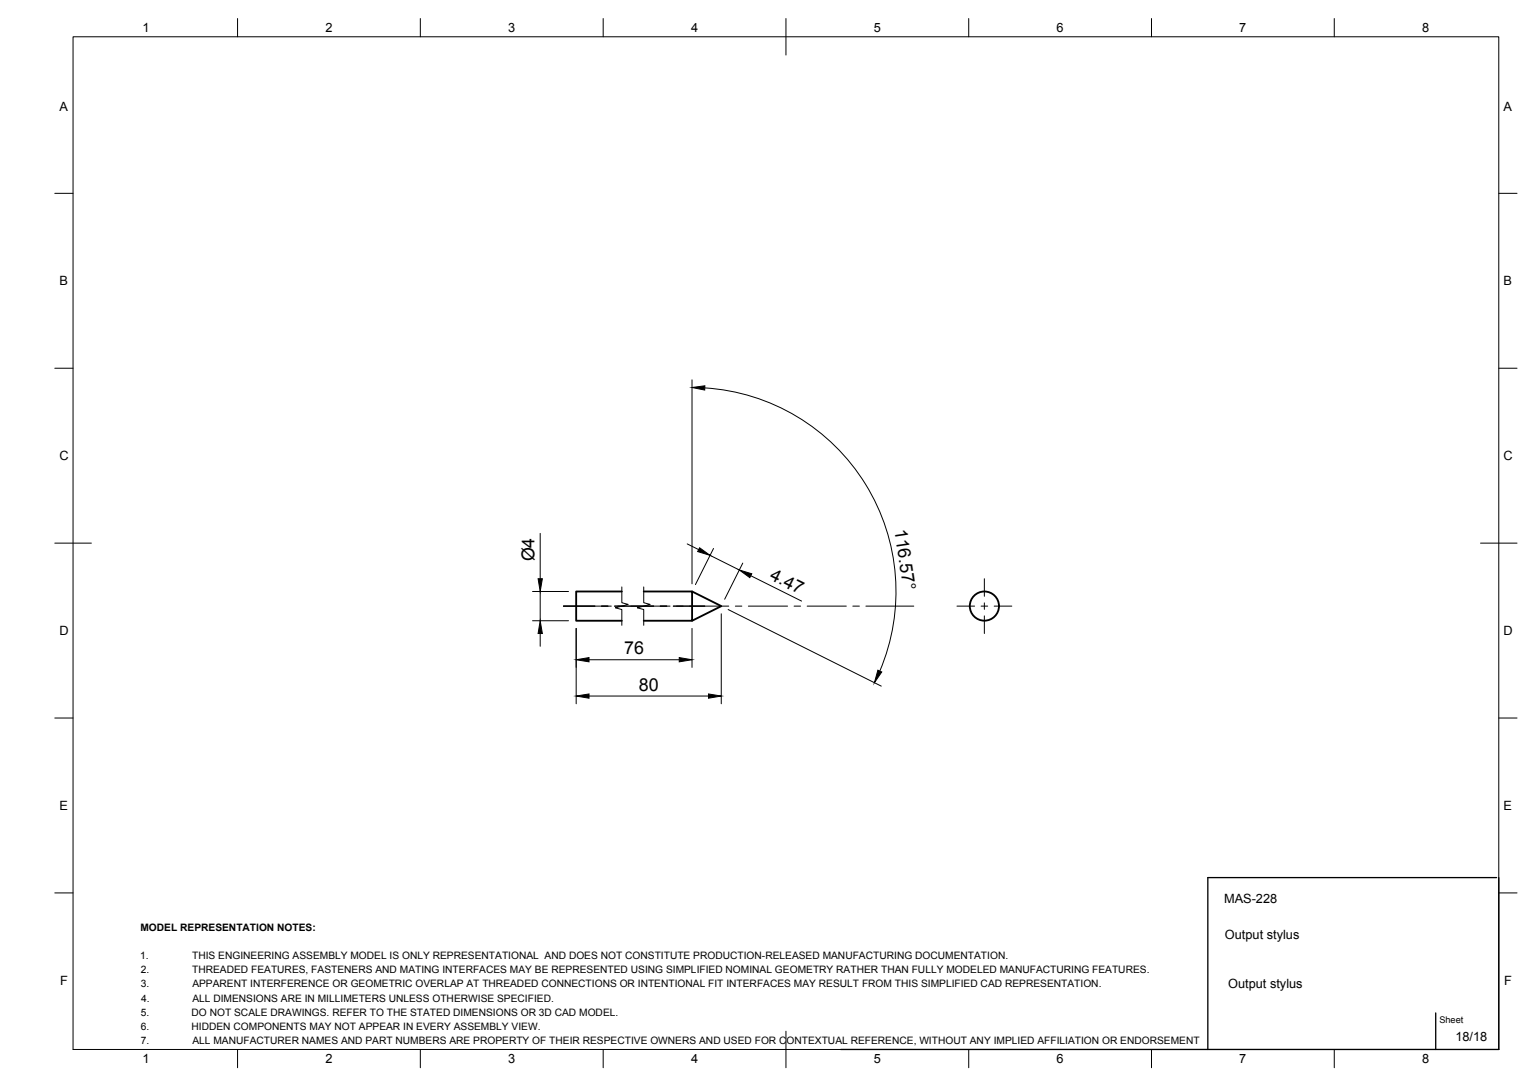
ISO-10303-21;
HEADER;
/* Generated by software containing ST-Developer
 * from STEP Tools, Inc. (www.steptools.com) 
 */

FILE_DESCRIPTION(
/* description */ ('Independent Peaucellier-Lipkin straight-line linkage. Radius arms 100
 mm, inversion-cell links 60 mm, crank radius and fixed-pivot spacing 
32 mm. Inversion constant 6400 mm squared, nominal output straight lin
e X=100 mm. Overhead bearing bridge clears the layered moving links. N
o accuracy or load rating assigned.'),
/* implementation_level */ '2;1');

FILE_NAME(
/* name */ 'Output stylus.step',
/* time_stamp */ '2026-11-09T18:06:16-08:00',
/* author */ (''),
/* organization */ (''),
/* preprocessor_version */ 'ST-DEVELOPER v20.2',
/* originating_system */ 'Autodesk Translation Framework v15.17.0.0',
/* authorisation */ '');

FILE_SCHEMA (('AUTOMOTIVE_DESIGN { 1 0 10303 214 3 1 1 }'));
ENDSEC;

DATA;
#10=MECHANICAL_DESIGN_GEOMETRIC_PRESENTATION_REPRESENTATION('',(#294),#3581);
#247=CONICAL_SURFACE('',#2252,1.,0.463647609000806);
#260=SHAPE_REPRESENTATION_RELATIONSHIP('SRR','None',#3694,#277);
#277=ADVANCED_BREP_SHAPE_REPRESENTATION('',(#311),#3576);
#294=STYLED_ITEM('',(#3785),#311);
#311=MANIFOLD_SOLID_BREP('Body1',#1880);
#411=PLANE('',#2251);
#510=FACE_OUTER_BOUND('',#662,.T.);
#511=FACE_OUTER_BOUND('',#663,.T.);
#512=FACE_OUTER_BOUND('',#664,.T.);
#662=EDGE_LOOP('',(#1628,#1629,#1630,#1631));
#663=EDGE_LOOP('',(#1632));
#664=EDGE_LOOP('',(#1633,#1634,#1635));
#775=LINE('',#3392,#873);
#776=LINE('',#3397,#874);
#873=VECTOR('',#2793,2.);
#874=VECTOR('',#2800,1.);
#967=CIRCLE('',#2249,2.);
#968=CIRCLE('',#2250,2.);
#1093=VERTEX_POINT('',#3389);
#1094=VERTEX_POINT('',#3391);
#1095=VERTEX_POINT('',#3396);
#1276=EDGE_CURVE('',#1093,#1093,#967,.T.);
#1277=EDGE_CURVE('',#1093,#1094,#775,.T.);
#1278=EDGE_CURVE('',#1094,#1094,#968,.T.);
#1279=EDGE_CURVE('',#1094,#1095,#776,.T.);
#1628=ORIENTED_EDGE('',*,*,#1276,.F.);
#1629=ORIENTED_EDGE('',*,*,#1277,.T.);
#1630=ORIENTED_EDGE('',*,*,#1278,.T.);
#1631=ORIENTED_EDGE('',*,*,#1277,.F.);
#1632=ORIENTED_EDGE('',*,*,#1276,.T.);
#1633=ORIENTED_EDGE('',*,*,#1278,.F.);
#1634=ORIENTED_EDGE('',*,*,#1279,.T.);
#1635=ORIENTED_EDGE('',*,*,#1279,.F.);
#1746=CYLINDRICAL_SURFACE('',#2248,2.);
#1842=ADVANCED_FACE('',(#510),#1746,.T.);
#1843=ADVANCED_FACE('',(#511),#411,.T.);
#1844=ADVANCED_FACE('',(#512),#247,.T.);
#1880=CLOSED_SHELL('',(#1842,#1843,#1844));
#2247=AXIS2_PLACEMENT_3D('',#3387,#2787,#2788);
#2248=AXIS2_PLACEMENT_3D('',#3388,#2789,#2790);
#2249=AXIS2_PLACEMENT_3D('',#3390,#2791,#2792);
#2250=AXIS2_PLACEMENT_3D('',#3393,#2794,#2795);
#2251=AXIS2_PLACEMENT_3D('',#3394,#2796,#2797);
#2252=AXIS2_PLACEMENT_3D('',#3395,#2798,#2799);
#2787=DIRECTION('axis',(0.,0.,1.));
#2788=DIRECTION('refdir',(1.,0.,0.));
#2789=DIRECTION('center_axis',(0.,0.,1.));
#2790=DIRECTION('ref_axis',(1.,0.,0.));
#2791=DIRECTION('center_axis',(0.,0.,1.));
#2792=DIRECTION('ref_axis',(1.,0.,0.));
#2793=DIRECTION('',(0.,0.,-1.));
#2794=DIRECTION('center_axis',(0.,0.,1.));
#2795=DIRECTION('ref_axis',(1.,0.,0.));
#2796=DIRECTION('center_axis',(0.,0.,1.));
#2797=DIRECTION('ref_axis',(1.,0.,0.));
#2798=DIRECTION('center_axis',(0.,0.,1.));
#2799=DIRECTION('ref_axis',(1.,0.,0.));
#2800=DIRECTION('',(0.447213595499958,5.47678698264203E-17,-0.894427190999916));
#3387=CARTESIAN_POINT('',(0.,0.,0.));
#3388=CARTESIAN_POINT('Origin',(0.,0.,4.));
#3389=CARTESIAN_POINT('',(-2.,-2.44929359829471E-16,80.));
#3390=CARTESIAN_POINT('Origin',(0.,0.,80.));
#3391=CARTESIAN_POINT('',(-2.,-2.44929359829471E-16,4.));
#3392=CARTESIAN_POINT('',(-2.,-2.44929359829471E-16,4.));
#3393=CARTESIAN_POINT('Origin',(0.,0.,4.));
#3394=CARTESIAN_POINT('Origin',(0.,0.,80.));
#3395=CARTESIAN_POINT('Origin',(0.,0.,2.));
#3396=CARTESIAN_POINT('',(0.,0.,0.));
#3397=CARTESIAN_POINT('',(-1.,-1.22464679914735E-16,2.));
#3557=UNCERTAINTY_MEASURE_WITH_UNIT(LENGTH_MEASURE(0.01),#3582,
'DISTANCE_ACCURACY_VALUE',
'Maximum model space distance between geometric entities at asserted c
onnectivities');
#3562=UNCERTAINTY_MEASURE_WITH_UNIT(LENGTH_MEASURE(0.01),#3582,
'DISTANCE_ACCURACY_VALUE',
'Maximum model space distance between geometric entities at asserted c
onnectivities');
#3576=(
GEOMETRIC_REPRESENTATION_CONTEXT(3)
GLOBAL_UNCERTAINTY_ASSIGNED_CONTEXT((#3557))
GLOBAL_UNIT_ASSIGNED_CONTEXT((#3582,#3584,#3585))
REPRESENTATION_CONTEXT('','3D')
);
#3581=(
GEOMETRIC_REPRESENTATION_CONTEXT(3)
GLOBAL_UNCERTAINTY_ASSIGNED_CONTEXT((#3562))
GLOBAL_UNIT_ASSIGNED_CONTEXT((#3582,#3584,#3585))
REPRESENTATION_CONTEXT('','3D')
);
#3582=(
LENGTH_UNIT()
NAMED_UNIT(*)
SI_UNIT(.MILLI.,.METRE.)
);
#3584=(
NAMED_UNIT(*)
PLANE_ANGLE_UNIT()
SI_UNIT($,.RADIAN.)
);
#3585=(
NAMED_UNIT(*)
SI_UNIT($,.STERADIAN.)
SOLID_ANGLE_UNIT()
);
#3599=SHAPE_DEFINITION_REPRESENTATION(#3617,#3694);
#3617=PRODUCT_DEFINITION_SHAPE('',$,#3713);
#3694=SHAPE_REPRESENTATION('',(#2247),#3576);
#3699=PRODUCT_DEFINITION_CONTEXT('part definition',#3755,'design');
#3713=PRODUCT_DEFINITION('Output stylus','Output stylus',#3731,#3699);
#3731=PRODUCT_DEFINITION_FORMATION('',$,#3770);
#3755=APPLICATION_CONTEXT(
'Core Data for Automotive Mechanical Design Process');
#3756=PRODUCT_CONTEXT('part definition',#3755,'mechanical');
#3770=PRODUCT('Output stylus','Output stylus',$,(#3756));
#3785=PRESENTATION_STYLE_ASSIGNMENT((#3798));
#3798=SURFACE_STYLE_USAGE(.BOTH.,#3811);
#3811=SURFACE_SIDE_STYLE('',(#3824));
#3824=SURFACE_STYLE_FILL_AREA(#3837);
#3837=FILL_AREA_STYLE('Stylus light gray',(#3850));
#3850=FILL_AREA_STYLE_COLOUR('Stylus light gray',#3863);
#3863=COLOUR_RGB('Stylus light gray',0.725490196078431,0.752941176470588,
0.792156862745098);
ENDSEC;
END-ISO-10303-21;
